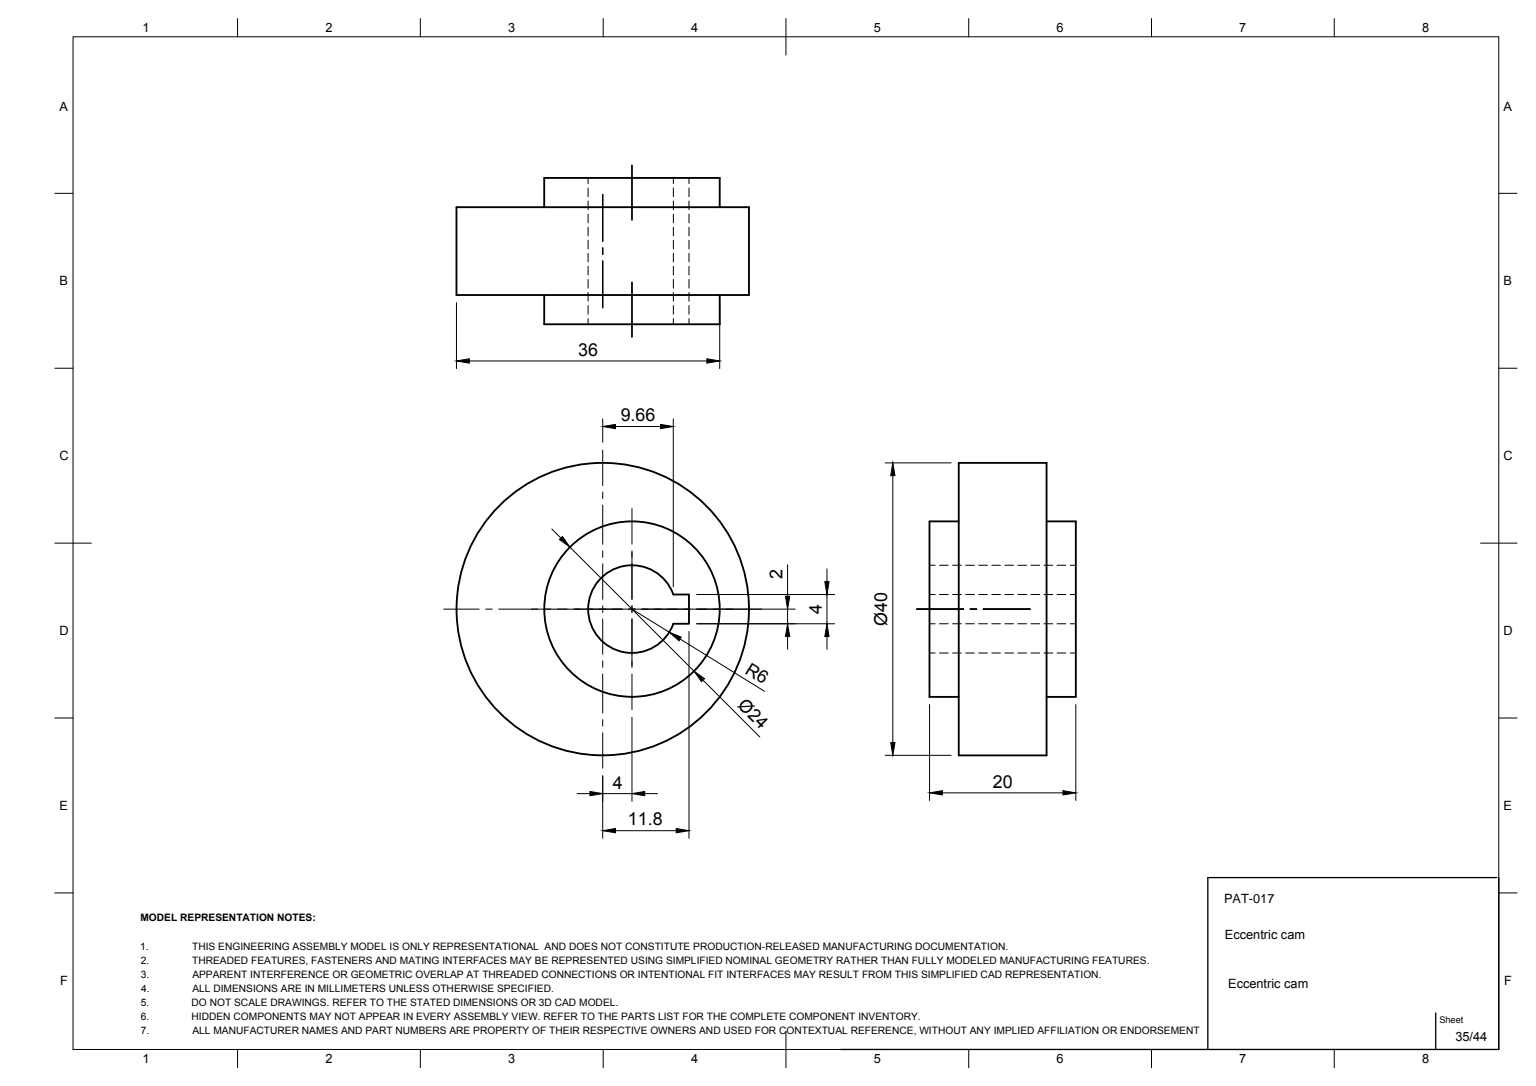
ISO-10303-21;
HEADER;
/* Generated by software containing ST-Developer
 * from STEP Tools, Inc. (www.steptools.com) 
 */

FILE_DESCRIPTION(
/* description */ ('Cam-and-follower valve demonstrator'),
/* implementation_level */ '2;1');

FILE_NAME(
/* name */ 'Eccentric cam.step',
/* time_stamp */ '2026-10-28T03:25:17-07:00',
/* author */ (''),
/* organization */ (''),
/* preprocessor_version */ 'ST-DEVELOPER v20.2',
/* originating_system */ 'Autodesk Translation Framework v15.17.0.0',
/* authorisation */ '');

FILE_SCHEMA (('AUTOMOTIVE_DESIGN { 1 0 10303 214 3 1 1 }'));
ENDSEC;

DATA;
#10=MECHANICAL_DESIGN_GEOMETRIC_PRESENTATION_REPRESENTATION('',(#445),#12896);
#366=SHAPE_REPRESENTATION_RELATIONSHIP('SRR','None',#13085,#402);
#402=ADVANCED_BREP_SHAPE_REPRESENTATION('',(#486),#12885);
#445=STYLED_ITEM('',(#13344),#486);
#486=MANIFOLD_SOLID_BREP('Body1',#6214);
#638=FACE_BOUND('',#1896,.T.);
#639=FACE_BOUND('',#1901,.T.);
#640=FACE_BOUND('',#1904,.T.);
#641=FACE_BOUND('',#1906,.T.);
#923=CIRCLE('',#7214,1.2);
#924=CIRCLE('',#7215,0.6);
#925=CIRCLE('',#7217,0.6);
#926=CIRCLE('',#7219,1.2);
#927=CIRCLE('',#7220,1.2);
#928=CIRCLE('',#7222,1.2);
#929=CIRCLE('',#7225,2.);
#930=CIRCLE('',#7226,2.);
#1073=CYLINDRICAL_SURFACE('',#7216,0.6);
#1074=CYLINDRICAL_SURFACE('',#7218,1.2);
#1075=CYLINDRICAL_SURFACE('',#7221,1.2);
#1076=CYLINDRICAL_SURFACE('',#7224,2.);
#1381=FACE_OUTER_BOUND('',#1892,.T.);
#1382=FACE_OUTER_BOUND('',#1893,.T.);
#1383=FACE_OUTER_BOUND('',#1894,.T.);
#1384=FACE_OUTER_BOUND('',#1895,.T.);
#1385=FACE_OUTER_BOUND('',#1897,.T.);
#1386=FACE_OUTER_BOUND('',#1898,.T.);
#1387=FACE_OUTER_BOUND('',#1899,.T.);
#1388=FACE_OUTER_BOUND('',#1900,.T.);
#1389=FACE_OUTER_BOUND('',#1902,.T.);
#1390=FACE_OUTER_BOUND('',#1903,.T.);
#1391=FACE_OUTER_BOUND('',#1905,.T.);
#1892=EDGE_LOOP('',(#5287,#5288,#5289,#5290));
#1893=EDGE_LOOP('',(#5291,#5292,#5293,#5294));
#1894=EDGE_LOOP('',(#5295,#5296,#5297,#5298));
#1895=EDGE_LOOP('',(#5299));
#1896=EDGE_LOOP('',(#5300,#5301,#5302,#5303));
#1897=EDGE_LOOP('',(#5304,#5305,#5306,#5307));
#1898=EDGE_LOOP('',(#5308,#5309,#5310,#5311));
#1899=EDGE_LOOP('',(#5312,#5313,#5314,#5315));
#1900=EDGE_LOOP('',(#5316));
#1901=EDGE_LOOP('',(#5317,#5318,#5319,#5320));
#1902=EDGE_LOOP('',(#5321,#5322,#5323,#5324));
#1903=EDGE_LOOP('',(#5325));
#1904=EDGE_LOOP('',(#5326));
#1905=EDGE_LOOP('',(#5327));
#1906=EDGE_LOOP('',(#5328));
#2312=LINE('',#12403,#2734);
#2313=LINE('',#12405,#2735);
#2314=LINE('',#12407,#2736);
#2315=LINE('',#12408,#2737);
#2316=LINE('',#12411,#2738);
#2317=LINE('',#12413,#2739);
#2318=LINE('',#12414,#2740);
#2319=LINE('',#12417,#2741);
#2320=LINE('',#12419,#2742);
#2321=LINE('',#12420,#2743);
#2322=LINE('',#12431,#2744);
#2323=LINE('',#12435,#2745);
#2324=LINE('',#12442,#2746);
#2734=VECTOR('',#8909,1.);
#2735=VECTOR('',#8910,1.);
#2736=VECTOR('',#8911,1.);
#2737=VECTOR('',#8912,1.);
#2738=VECTOR('',#8915,1.);
#2739=VECTOR('',#8916,1.);
#2740=VECTOR('',#8917,1.);
#2741=VECTOR('',#8920,1.);
#2742=VECTOR('',#8921,1.);
#2743=VECTOR('',#8922,1.);
#2744=VECTOR('',#8937,1.2);
#2745=VECTOR('',#8942,1.2);
#2746=VECTOR('',#8951,2.);
#3242=VERTEX_POINT('',#12401);
#3243=VERTEX_POINT('',#12402);
#3244=VERTEX_POINT('',#12404);
#3245=VERTEX_POINT('',#12406);
#3246=VERTEX_POINT('',#12410);
#3247=VERTEX_POINT('',#12412);
#3248=VERTEX_POINT('',#12416);
#3249=VERTEX_POINT('',#12418);
#3250=VERTEX_POINT('',#12422);
#3251=VERTEX_POINT('',#12428);
#3252=VERTEX_POINT('',#12430);
#3253=VERTEX_POINT('',#12434);
#3254=VERTEX_POINT('',#12439);
#3255=VERTEX_POINT('',#12441);
#3940=EDGE_CURVE('',#3242,#3243,#2312,.T.);
#3941=EDGE_CURVE('',#3242,#3244,#2313,.T.);
#3942=EDGE_CURVE('',#3245,#3244,#2314,.T.);
#3943=EDGE_CURVE('',#3243,#3245,#2315,.T.);
#3944=EDGE_CURVE('',#3246,#3242,#2316,.T.);
#3945=EDGE_CURVE('',#3246,#3247,#2317,.T.);
#3946=EDGE_CURVE('',#3244,#3247,#2318,.T.);
#3947=EDGE_CURVE('',#3248,#3246,#2319,.T.);
#3948=EDGE_CURVE('',#3249,#3248,#2320,.T.);
#3949=EDGE_CURVE('',#3247,#3249,#2321,.T.);
#3950=EDGE_CURVE('',#3250,#3250,#923,.T.);
#3951=EDGE_CURVE('',#3249,#3245,#924,.T.);
#3952=EDGE_CURVE('',#3243,#3248,#925,.T.);
#3953=EDGE_CURVE('',#3251,#3251,#926,.T.);
#3954=EDGE_CURVE('',#3251,#3252,#2322,.T.);
#3955=EDGE_CURVE('',#3252,#3252,#927,.T.);
#3956=EDGE_CURVE('',#3250,#3253,#2323,.T.);
#3957=EDGE_CURVE('',#3253,#3253,#928,.T.);
#3958=EDGE_CURVE('',#3254,#3254,#929,.T.);
#3959=EDGE_CURVE('',#3254,#3255,#2324,.T.);
#3960=EDGE_CURVE('',#3255,#3255,#930,.T.);
#5287=ORIENTED_EDGE('',*,*,#3940,.F.);
#5288=ORIENTED_EDGE('',*,*,#3941,.T.);
#5289=ORIENTED_EDGE('',*,*,#3942,.F.);
#5290=ORIENTED_EDGE('',*,*,#3943,.F.);
#5291=ORIENTED_EDGE('',*,*,#3944,.F.);
#5292=ORIENTED_EDGE('',*,*,#3945,.T.);
#5293=ORIENTED_EDGE('',*,*,#3946,.F.);
#5294=ORIENTED_EDGE('',*,*,#3941,.F.);
#5295=ORIENTED_EDGE('',*,*,#3947,.F.);
#5296=ORIENTED_EDGE('',*,*,#3948,.F.);
#5297=ORIENTED_EDGE('',*,*,#3949,.F.);
#5298=ORIENTED_EDGE('',*,*,#3945,.F.);
#5299=ORIENTED_EDGE('',*,*,#3950,.T.);
#5300=ORIENTED_EDGE('',*,*,#3942,.T.);
#5301=ORIENTED_EDGE('',*,*,#3946,.T.);
#5302=ORIENTED_EDGE('',*,*,#3949,.T.);
#5303=ORIENTED_EDGE('',*,*,#3951,.T.);
#5304=ORIENTED_EDGE('',*,*,#3943,.T.);
#5305=ORIENTED_EDGE('',*,*,#3951,.F.);
#5306=ORIENTED_EDGE('',*,*,#3948,.T.);
#5307=ORIENTED_EDGE('',*,*,#3952,.F.);
#5308=ORIENTED_EDGE('',*,*,#3953,.F.);
#5309=ORIENTED_EDGE('',*,*,#3954,.T.);
#5310=ORIENTED_EDGE('',*,*,#3955,.T.);
#5311=ORIENTED_EDGE('',*,*,#3954,.F.);
#5312=ORIENTED_EDGE('',*,*,#3950,.F.);
#5313=ORIENTED_EDGE('',*,*,#3956,.T.);
#5314=ORIENTED_EDGE('',*,*,#3957,.F.);
#5315=ORIENTED_EDGE('',*,*,#3956,.F.);
#5316=ORIENTED_EDGE('',*,*,#3955,.F.);
#5317=ORIENTED_EDGE('',*,*,#3940,.T.);
#5318=ORIENTED_EDGE('',*,*,#3952,.T.);
#5319=ORIENTED_EDGE('',*,*,#3947,.T.);
#5320=ORIENTED_EDGE('',*,*,#3944,.T.);
#5321=ORIENTED_EDGE('',*,*,#3958,.F.);
#5322=ORIENTED_EDGE('',*,*,#3959,.T.);
#5323=ORIENTED_EDGE('',*,*,#3960,.T.);
#5324=ORIENTED_EDGE('',*,*,#3959,.F.);
#5325=ORIENTED_EDGE('',*,*,#3958,.T.);
#5326=ORIENTED_EDGE('',*,*,#3957,.T.);
#5327=ORIENTED_EDGE('',*,*,#3960,.F.);
#5328=ORIENTED_EDGE('',*,*,#3953,.T.);
#5755=PLANE('',#7210);
#5756=PLANE('',#7211);
#5757=PLANE('',#7212);
#5758=PLANE('',#7213);
#5759=PLANE('',#7223);
#5760=PLANE('',#7227);
#5761=PLANE('',#7228);
#6097=ADVANCED_FACE('',(#1381),#5755,.F.);
#6098=ADVANCED_FACE('',(#1382),#5756,.F.);
#6099=ADVANCED_FACE('',(#1383),#5757,.F.);
#6100=ADVANCED_FACE('',(#1384,#638),#5758,.T.);
#6101=ADVANCED_FACE('',(#1385),#1073,.F.);
#6102=ADVANCED_FACE('',(#1386),#1074,.T.);
#6103=ADVANCED_FACE('',(#1387),#1075,.T.);
#6104=ADVANCED_FACE('',(#1388,#639),#5759,.F.);
#6105=ADVANCED_FACE('',(#1389),#1076,.T.);
#6106=ADVANCED_FACE('',(#1390,#640),#5760,.T.);
#6107=ADVANCED_FACE('',(#1391,#641),#5761,.F.);
#6214=CLOSED_SHELL('',(#6097,#6098,#6099,#6100,#6101,#6102,#6103,#6104,
#6105,#6106,#6107));
#7209=AXIS2_PLACEMENT_3D('',#12399,#8905,#8906);
#7210=AXIS2_PLACEMENT_3D('',#12400,#8907,#8908);
#7211=AXIS2_PLACEMENT_3D('',#12409,#8913,#8914);
#7212=AXIS2_PLACEMENT_3D('',#12415,#8918,#8919);
#7213=AXIS2_PLACEMENT_3D('',#12421,#8923,#8924);
#7214=AXIS2_PLACEMENT_3D('',#12423,#8925,#8926);
#7215=AXIS2_PLACEMENT_3D('',#12424,#8927,#8928);
#7216=AXIS2_PLACEMENT_3D('',#12425,#8929,#8930);
#7217=AXIS2_PLACEMENT_3D('',#12426,#8931,#8932);
#7218=AXIS2_PLACEMENT_3D('',#12427,#8933,#8934);
#7219=AXIS2_PLACEMENT_3D('',#12429,#8935,#8936);
#7220=AXIS2_PLACEMENT_3D('',#12432,#8938,#8939);
#7221=AXIS2_PLACEMENT_3D('',#12433,#8940,#8941);
#7222=AXIS2_PLACEMENT_3D('',#12436,#8943,#8944);
#7223=AXIS2_PLACEMENT_3D('',#12437,#8945,#8946);
#7224=AXIS2_PLACEMENT_3D('',#12438,#8947,#8948);
#7225=AXIS2_PLACEMENT_3D('',#12440,#8949,#8950);
#7226=AXIS2_PLACEMENT_3D('',#12443,#8952,#8953);
#7227=AXIS2_PLACEMENT_3D('',#12444,#8954,#8955);
#7228=AXIS2_PLACEMENT_3D('',#12445,#8956,#8957);
#8905=DIRECTION('axis',(0.,0.,1.));
#8906=DIRECTION('refdir',(1.,0.,0.));
#8907=DIRECTION('center_axis',(-1.,0.,0.));
#8908=DIRECTION('ref_axis',(0.,0.,1.));
#8909=DIRECTION('',(0.,0.,1.));
#8910=DIRECTION('',(0.,1.,0.));
#8911=DIRECTION('',(0.,0.,-1.));
#8912=DIRECTION('',(0.,1.,0.));
#8913=DIRECTION('center_axis',(0.,0.,-1.));
#8914=DIRECTION('ref_axis',(-1.,0.,0.));
#8915=DIRECTION('',(-1.,0.,0.));
#8916=DIRECTION('',(0.,1.,0.));
#8917=DIRECTION('',(1.,0.,0.));
#8918=DIRECTION('center_axis',(1.,0.,0.));
#8919=DIRECTION('ref_axis',(0.,0.,-1.));
#8920=DIRECTION('',(0.,0.,-1.));
#8921=DIRECTION('',(0.,-1.,0.));
#8922=DIRECTION('',(0.,0.,1.));
#8923=DIRECTION('center_axis',(0.,1.,0.));
#8924=DIRECTION('ref_axis',(1.,0.,0.));
#8925=DIRECTION('center_axis',(0.,1.,0.));
#8926=DIRECTION('ref_axis',(1.,0.,0.));
#8927=DIRECTION('center_axis',(0.,-1.,0.));
#8928=DIRECTION('ref_axis',(1.,0.,0.));
#8929=DIRECTION('center_axis',(0.,1.,0.));
#8930=DIRECTION('ref_axis',(-1.83697019872103E-16,0.,1.));
#8931=DIRECTION('center_axis',(0.,1.,0.));
#8932=DIRECTION('ref_axis',(1.,0.,0.));
#8933=DIRECTION('center_axis',(0.,1.,0.));
#8934=DIRECTION('ref_axis',(1.,0.,0.));
#8935=DIRECTION('center_axis',(0.,1.,0.));
#8936=DIRECTION('ref_axis',(1.,0.,0.));
#8937=DIRECTION('',(0.,-1.,0.));
#8938=DIRECTION('center_axis',(0.,1.,0.));
#8939=DIRECTION('ref_axis',(1.,0.,0.));
#8940=DIRECTION('center_axis',(0.,1.,0.));
#8941=DIRECTION('ref_axis',(1.,0.,0.));
#8942=DIRECTION('',(0.,-1.,0.));
#8943=DIRECTION('center_axis',(0.,-1.,0.));
#8944=DIRECTION('ref_axis',(1.,0.,0.));
#8945=DIRECTION('center_axis',(0.,1.,0.));
#8946=DIRECTION('ref_axis',(1.,0.,0.));
#8947=DIRECTION('center_axis',(0.,1.,0.));
#8948=DIRECTION('ref_axis',(1.,0.,0.));
#8949=DIRECTION('center_axis',(0.,1.,0.));
#8950=DIRECTION('ref_axis',(1.,0.,0.));
#8951=DIRECTION('',(0.,-1.,0.));
#8952=DIRECTION('center_axis',(0.,1.,0.));
#8953=DIRECTION('ref_axis',(1.,0.,0.));
#8954=DIRECTION('center_axis',(0.,1.,0.));
#8955=DIRECTION('ref_axis',(1.,0.,0.));
#8956=DIRECTION('center_axis',(0.,1.,0.));
#8957=DIRECTION('ref_axis',(1.,0.,0.));
#12399=CARTESIAN_POINT('',(0.,0.,0.));
#12400=CARTESIAN_POINT('Origin',(-0.2,-1.1,3.22));
#12401=CARTESIAN_POINT('',(-0.2,-1.,3.22));
#12402=CARTESIAN_POINT('',(-0.2,-1.,3.43431457505076));
#12403=CARTESIAN_POINT('',(-0.2,-1.,3.61));
#12404=CARTESIAN_POINT('',(-0.2,1.,3.22));
#12405=CARTESIAN_POINT('',(-0.2,-1.1,3.22));
#12406=CARTESIAN_POINT('',(-0.2,1.,3.43431457505076));
#12407=CARTESIAN_POINT('',(-0.2,1.,3.61));
#12408=CARTESIAN_POINT('',(-0.2,-1.1,3.43431457505076));
#12409=CARTESIAN_POINT('Origin',(0.2,-1.1,3.22));
#12410=CARTESIAN_POINT('',(0.2,-1.,3.22));
#12411=CARTESIAN_POINT('',(0.1,-1.,3.22));
#12412=CARTESIAN_POINT('',(0.2,1.,3.22));
#12413=CARTESIAN_POINT('',(0.2,-1.1,3.22));
#12414=CARTESIAN_POINT('',(0.1,1.,3.22));
#12415=CARTESIAN_POINT('Origin',(0.2,-1.1,4.));
#12416=CARTESIAN_POINT('',(0.2,-1.,3.43431457505076));
#12417=CARTESIAN_POINT('',(0.2,-1.,4.));
#12418=CARTESIAN_POINT('',(0.2,1.,3.43431457505076));
#12419=CARTESIAN_POINT('',(0.2,-1.1,3.43431457505076));
#12420=CARTESIAN_POINT('',(0.2,1.,4.));
#12421=CARTESIAN_POINT('Origin',(0.,1.,4.));
#12422=CARTESIAN_POINT('',(-1.2,1.,4.));
#12423=CARTESIAN_POINT('Origin',(0.,1.,4.));
#12424=CARTESIAN_POINT('Origin',(0.,1.,4.));
#12425=CARTESIAN_POINT('Origin',(0.,-1.1,4.));
#12426=CARTESIAN_POINT('Origin',(0.,-1.,4.));
#12427=CARTESIAN_POINT('Origin',(0.,-1.,4.));
#12428=CARTESIAN_POINT('',(-1.2,-0.6,4.));
#12429=CARTESIAN_POINT('Origin',(0.,-0.6,4.));
#12430=CARTESIAN_POINT('',(-1.2,-1.,4.));
#12431=CARTESIAN_POINT('',(-1.2,-1.,4.));
#12432=CARTESIAN_POINT('Origin',(0.,-1.,4.));
#12433=CARTESIAN_POINT('Origin',(0.,-1.,4.));
#12434=CARTESIAN_POINT('',(-1.2,0.6,4.));
#12435=CARTESIAN_POINT('',(-1.2,-1.,4.));
#12436=CARTESIAN_POINT('Origin',(0.,0.6,4.));
#12437=CARTESIAN_POINT('Origin',(0.,-1.,4.));
#12438=CARTESIAN_POINT('Origin',(0.,-0.6,4.4));
#12439=CARTESIAN_POINT('',(-2.,0.6,4.4));
#12440=CARTESIAN_POINT('Origin',(0.,0.6,4.4));
#12441=CARTESIAN_POINT('',(-2.,-0.6,4.4));
#12442=CARTESIAN_POINT('',(-2.,-0.6,4.4));
#12443=CARTESIAN_POINT('Origin',(0.,-0.6,4.4));
#12444=CARTESIAN_POINT('Origin',(0.,0.6,4.4));
#12445=CARTESIAN_POINT('Origin',(0.,-0.6,4.4));
#12842=UNCERTAINTY_MEASURE_WITH_UNIT(LENGTH_MEASURE(0.001),#12897,
'DISTANCE_ACCURACY_VALUE',
'Maximum model space distance between geometric entities at asserted c
onnectivities');
#12853=UNCERTAINTY_MEASURE_WITH_UNIT(LENGTH_MEASURE(0.001),#12897,
'DISTANCE_ACCURACY_VALUE',
'Maximum model space distance between geometric entities at asserted c
onnectivities');
#12885=(
GEOMETRIC_REPRESENTATION_CONTEXT(3)
GLOBAL_UNCERTAINTY_ASSIGNED_CONTEXT((#12842))
GLOBAL_UNIT_ASSIGNED_CONTEXT((#12897,#12899,#12900))
REPRESENTATION_CONTEXT('','3D')
);
#12896=(
GEOMETRIC_REPRESENTATION_CONTEXT(3)
GLOBAL_UNCERTAINTY_ASSIGNED_CONTEXT((#12853))
GLOBAL_UNIT_ASSIGNED_CONTEXT((#12897,#12899,#12900))
REPRESENTATION_CONTEXT('','3D')
);
#12897=(
LENGTH_UNIT()
NAMED_UNIT(*)
SI_UNIT(.CENTI.,.METRE.)
);
#12899=(
NAMED_UNIT(*)
PLANE_ANGLE_UNIT()
SI_UNIT($,.RADIAN.)
);
#12900=(
NAMED_UNIT(*)
SI_UNIT($,.STERADIAN.)
SOLID_ANGLE_UNIT()
);
#12932=SHAPE_DEFINITION_REPRESENTATION(#12981,#13085);
#12981=PRODUCT_DEFINITION_SHAPE('',$,#13128);
#13085=SHAPE_REPRESENTATION('',(#7209),#12885);
#13096=PRODUCT_DEFINITION_CONTEXT('part definition',#13224,'design');
#13128=PRODUCT_DEFINITION('Eccentric cam','Eccentric cam',#13170,#13096);
#13170=PRODUCT_DEFINITION_FORMATION('',$,#13257);
#13224=APPLICATION_CONTEXT(
'Core Data for Automotive Mechanical Design Process');
#13225=PRODUCT_CONTEXT('part definition',#13224,'mechanical');
#13257=PRODUCT('Eccentric cam','Eccentric cam','Eccentric cam',(#13225));
#13338=COLOUR_RGB('Off White',0.89,0.88,0.83);
#13339=FILL_AREA_STYLE_COLOUR('',#13338);
#13340=FILL_AREA_STYLE('',(#13339));
#13341=SURFACE_STYLE_FILL_AREA(#13340);
#13342=SURFACE_SIDE_STYLE('',(#13341));
#13343=SURFACE_STYLE_USAGE(.BOTH.,#13342);
#13344=PRESENTATION_STYLE_ASSIGNMENT((#13343));
ENDSEC;
END-ISO-10303-21;
